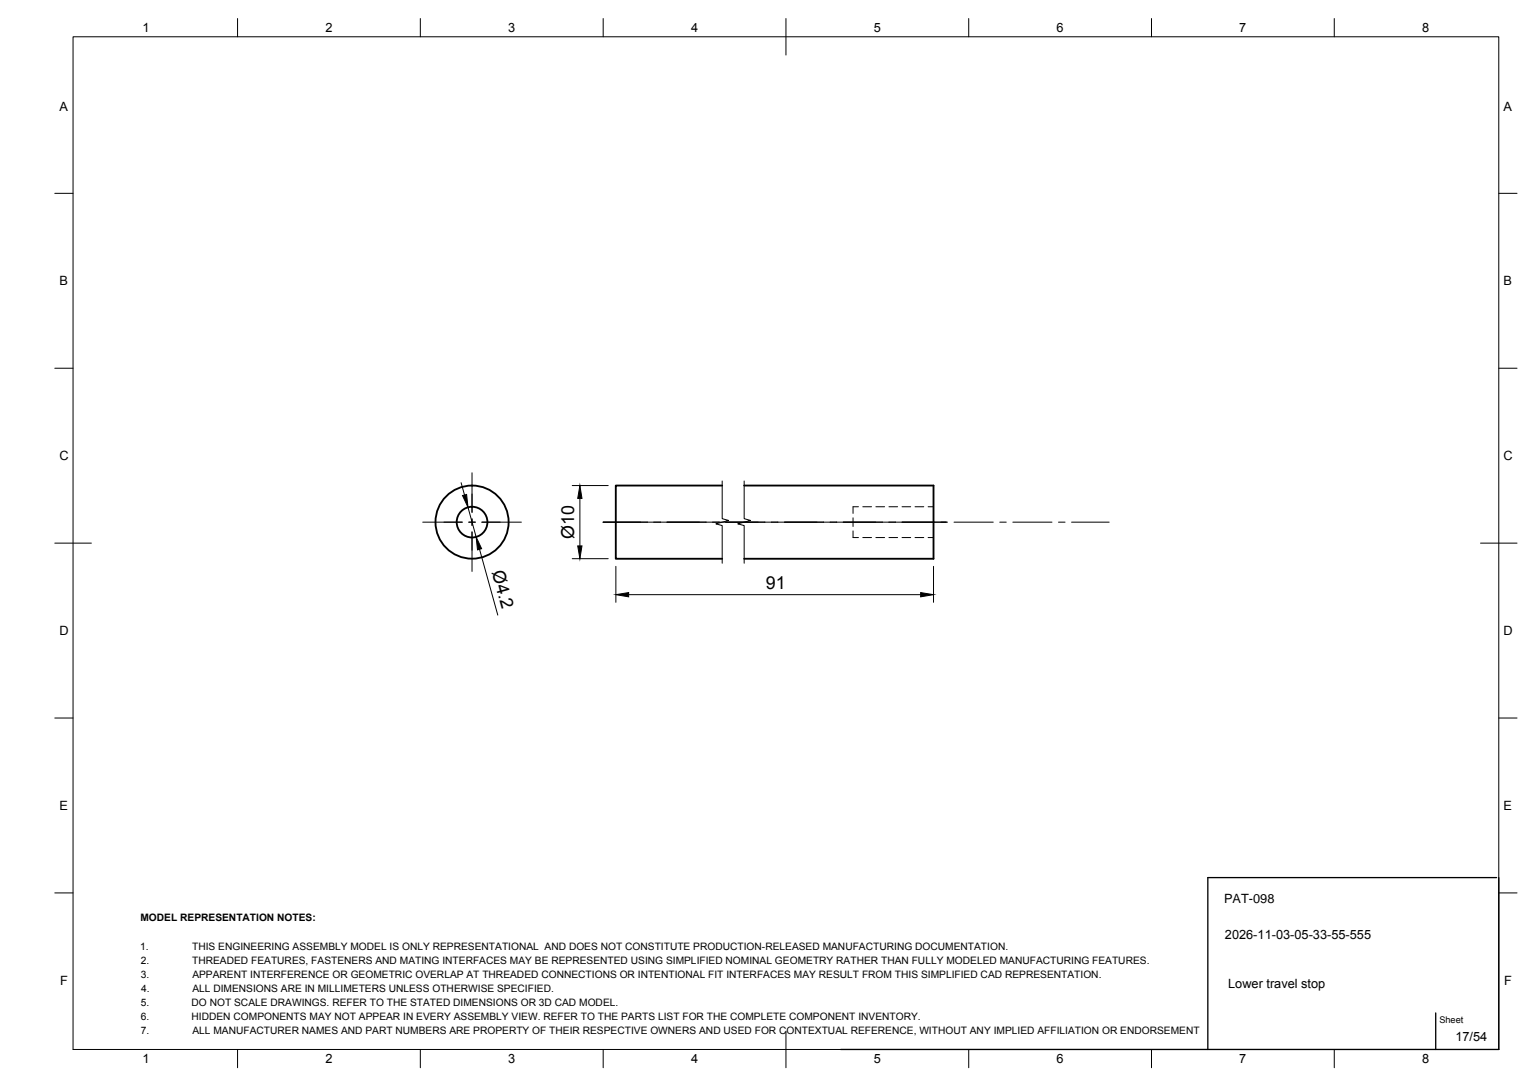
ISO-10303-21;
HEADER;
/* Generated by software containing ST-Developer
 * from STEP Tools, Inc. (www.steptools.com) 
 */

FILE_DESCRIPTION(
/* description */ ('Spring compression tester'),
/* implementation_level */ '2;1');

FILE_NAME(
/* name */ 'Lower travel stop.step',
/* time_stamp */ '2026-10-28T03:24:11-07:00',
/* author */ (''),
/* organization */ (''),
/* preprocessor_version */ 'ST-DEVELOPER v20.2',
/* originating_system */ 'Autodesk Translation Framework v15.17.0.0',
/* authorisation */ '');

FILE_SCHEMA (('AUTOMOTIVE_DESIGN { 1 0 10303 214 3 1 1 }'));
ENDSEC;

DATA;
#10=MECHANICAL_DESIGN_GEOMETRIC_PRESENTATION_REPRESENTATION('',(#1118),#43521);
#998=SHAPE_REPRESENTATION_RELATIONSHIP('SRR','None',#43810,#1058);
#1058=ADVANCED_BREP_SHAPE_REPRESENTATION('',(#1193),#43470);
#1118=STYLED_ITEM('',(#44188),#1193);
#1193=MANIFOLD_SOLID_BREP('Body1',#18555);
#1394=FACE_BOUND('',#3583,.T.);
#1710=PLANE('',#19712);
#1711=PLANE('',#19716);
#1712=PLANE('',#19717);
#2384=FACE_OUTER_BOUND('',#3578,.T.);
#2385=FACE_OUTER_BOUND('',#3579,.T.);
#2386=FACE_OUTER_BOUND('',#3580,.T.);
#2387=FACE_OUTER_BOUND('',#3581,.T.);
#2388=FACE_OUTER_BOUND('',#3582,.T.);
#3578=EDGE_LOOP('',(#13183,#13184,#13185,#13186));
#3579=EDGE_LOOP('',(#13187));
#3580=EDGE_LOOP('',(#13188,#13189,#13190,#13191));
#3581=EDGE_LOOP('',(#13192));
#3582=EDGE_LOOP('',(#13193));
#3583=EDGE_LOOP('',(#13194));
#4895=LINE('',#27492,#6327);
#4896=LINE('',#27499,#6328);
#6327=VECTOR('',#22339,0.21);
#6328=VECTOR('',#22348,0.5);
#7664=CIRCLE('',#19710,0.21);
#7665=CIRCLE('',#19711,0.21);
#7666=CIRCLE('',#19714,0.5);
#7667=CIRCLE('',#19715,0.5);
#8458=VERTEX_POINT('',#27489);
#8459=VERTEX_POINT('',#27491);
#8460=VERTEX_POINT('',#27496);
#8461=VERTEX_POINT('',#27498);
#10256=EDGE_CURVE('',#8458,#8458,#7664,.T.);
#10257=EDGE_CURVE('',#8458,#8459,#4895,.T.);
#10258=EDGE_CURVE('',#8459,#8459,#7665,.T.);
#10259=EDGE_CURVE('',#8460,#8460,#7666,.T.);
#10260=EDGE_CURVE('',#8460,#8461,#4896,.T.);
#10261=EDGE_CURVE('',#8461,#8461,#7667,.T.);
#13183=ORIENTED_EDGE('',*,*,#10256,.F.);
#13184=ORIENTED_EDGE('',*,*,#10257,.T.);
#13185=ORIENTED_EDGE('',*,*,#10258,.T.);
#13186=ORIENTED_EDGE('',*,*,#10257,.F.);
#13187=ORIENTED_EDGE('',*,*,#10258,.F.);
#13188=ORIENTED_EDGE('',*,*,#10259,.F.);
#13189=ORIENTED_EDGE('',*,*,#10260,.T.);
#13190=ORIENTED_EDGE('',*,*,#10261,.T.);
#13191=ORIENTED_EDGE('',*,*,#10260,.F.);
#13192=ORIENTED_EDGE('',*,*,#10259,.T.);
#13193=ORIENTED_EDGE('',*,*,#10261,.F.);
#13194=ORIENTED_EDGE('',*,*,#10256,.T.);
#17198=CYLINDRICAL_SURFACE('',#19709,0.21);
#17199=CYLINDRICAL_SURFACE('',#19713,0.5);
#17708=ADVANCED_FACE('',(#2384),#17198,.F.);
#17709=ADVANCED_FACE('',(#2385),#1710,.F.);
#17710=ADVANCED_FACE('',(#2386),#17199,.T.);
#17711=ADVANCED_FACE('',(#2387),#1711,.T.);
#17712=ADVANCED_FACE('',(#2388,#1394),#1712,.F.);
#18555=CLOSED_SHELL('',(#17708,#17709,#17710,#17711,#17712));
#19708=AXIS2_PLACEMENT_3D('',#27487,#22333,#22334);
#19709=AXIS2_PLACEMENT_3D('',#27488,#22335,#22336);
#19710=AXIS2_PLACEMENT_3D('',#27490,#22337,#22338);
#19711=AXIS2_PLACEMENT_3D('',#27493,#22340,#22341);
#19712=AXIS2_PLACEMENT_3D('',#27494,#22342,#22343);
#19713=AXIS2_PLACEMENT_3D('',#27495,#22344,#22345);
#19714=AXIS2_PLACEMENT_3D('',#27497,#22346,#22347);
#19715=AXIS2_PLACEMENT_3D('',#27500,#22349,#22350);
#19716=AXIS2_PLACEMENT_3D('',#27501,#22351,#22352);
#19717=AXIS2_PLACEMENT_3D('',#27502,#22353,#22354);
#22333=DIRECTION('axis',(0.,0.,1.));
#22334=DIRECTION('refdir',(1.,0.,0.));
#22335=DIRECTION('center_axis',(0.,0.,1.));
#22336=DIRECTION('ref_axis',(1.,0.,0.));
#22337=DIRECTION('center_axis',(0.,0.,1.));
#22338=DIRECTION('ref_axis',(1.,0.,0.));
#22339=DIRECTION('',(0.,0.,1.));
#22340=DIRECTION('center_axis',(0.,0.,1.));
#22341=DIRECTION('ref_axis',(1.,0.,0.));
#22342=DIRECTION('center_axis',(0.,0.,1.));
#22343=DIRECTION('ref_axis',(1.,0.,0.));
#22344=DIRECTION('center_axis',(0.,0.,1.));
#22345=DIRECTION('ref_axis',(1.,0.,0.));
#22346=DIRECTION('center_axis',(0.,0.,1.));
#22347=DIRECTION('ref_axis',(1.,0.,0.));
#22348=DIRECTION('',(0.,0.,-1.));
#22349=DIRECTION('center_axis',(0.,0.,1.));
#22350=DIRECTION('ref_axis',(1.,0.,0.));
#22351=DIRECTION('center_axis',(0.,0.,1.));
#22352=DIRECTION('ref_axis',(1.,0.,0.));
#22353=DIRECTION('center_axis',(0.,0.,1.));
#22354=DIRECTION('ref_axis',(1.,0.,0.));
#27487=CARTESIAN_POINT('',(0.,0.,0.));
#27488=CARTESIAN_POINT('Origin',(-6.,5.,-0.1));
#27489=CARTESIAN_POINT('',(-6.21,5.,0.));
#27490=CARTESIAN_POINT('Origin',(-6.,5.,0.));
#27491=CARTESIAN_POINT('',(-6.21,5.,1.1));
#27492=CARTESIAN_POINT('',(-6.21,5.,-0.1));
#27493=CARTESIAN_POINT('Origin',(-6.,5.,1.1));
#27494=CARTESIAN_POINT('Origin',(-6.,5.,1.1));
#27495=CARTESIAN_POINT('Origin',(-6.,5.,0.));
#27496=CARTESIAN_POINT('',(-6.5,5.,9.1));
#27497=CARTESIAN_POINT('Origin',(-6.,5.,9.1));
#27498=CARTESIAN_POINT('',(-6.5,5.,0.));
#27499=CARTESIAN_POINT('',(-6.5,5.,0.));
#27500=CARTESIAN_POINT('Origin',(-6.,5.,0.));
#27501=CARTESIAN_POINT('Origin',(-6.,5.,9.1));
#27502=CARTESIAN_POINT('Origin',(-6.,5.,0.));
#43402=UNCERTAINTY_MEASURE_WITH_UNIT(LENGTH_MEASURE(0.001),#43522,
'DISTANCE_ACCURACY_VALUE',
'Maximum model space distance between geometric entities at asserted c
onnectivities');
#43453=UNCERTAINTY_MEASURE_WITH_UNIT(LENGTH_MEASURE(0.001),#43522,
'DISTANCE_ACCURACY_VALUE',
'Maximum model space distance between geometric entities at asserted c
onnectivities');
#43470=(
GEOMETRIC_REPRESENTATION_CONTEXT(3)
GLOBAL_UNCERTAINTY_ASSIGNED_CONTEXT((#43402))
GLOBAL_UNIT_ASSIGNED_CONTEXT((#43522,#43524,#43525))
REPRESENTATION_CONTEXT('','3D')
);
#43521=(
GEOMETRIC_REPRESENTATION_CONTEXT(3)
GLOBAL_UNCERTAINTY_ASSIGNED_CONTEXT((#43453))
GLOBAL_UNIT_ASSIGNED_CONTEXT((#43522,#43524,#43525))
REPRESENTATION_CONTEXT('','3D')
);
#43522=(
LENGTH_UNIT()
NAMED_UNIT(*)
SI_UNIT(.CENTI.,.METRE.)
);
#43524=(
NAMED_UNIT(*)
PLANE_ANGLE_UNIT()
SI_UNIT($,.RADIAN.)
);
#43525=(
NAMED_UNIT(*)
SI_UNIT($,.STERADIAN.)
SOLID_ANGLE_UNIT()
);
#43542=SHAPE_DEFINITION_REPRESENTATION(#43609,#43810);
#43609=PRODUCT_DEFINITION_SHAPE('',$,#43878);
#43810=SHAPE_REPRESENTATION('',(#19708),#43470);
#43861=PRODUCT_DEFINITION_CONTEXT('part definition',#44064,'design');
#43878=PRODUCT_DEFINITION('Lower travel stop','Lower travel stop',#43945,
#43861);
#43945=PRODUCT_DEFINITION_FORMATION('',$,#44082);
#44064=APPLICATION_CONTEXT(
'Core Data for Automotive Mechanical Design Process');
#44065=PRODUCT_CONTEXT('part definition',#44064,'mechanical');
#44082=PRODUCT('Lower travel stop','Lower travel stop',
'Lower travel stop',(#44065));
#44182=COLOUR_RGB('Light Blue',0.38,0.62,0.78);
#44183=FILL_AREA_STYLE_COLOUR('',#44182);
#44184=FILL_AREA_STYLE('',(#44183));
#44185=SURFACE_STYLE_FILL_AREA(#44184);
#44186=SURFACE_SIDE_STYLE('',(#44185));
#44187=SURFACE_STYLE_USAGE(.BOTH.,#44186);
#44188=PRESENTATION_STYLE_ASSIGNMENT((#44187));
ENDSEC;
END-ISO-10303-21;
